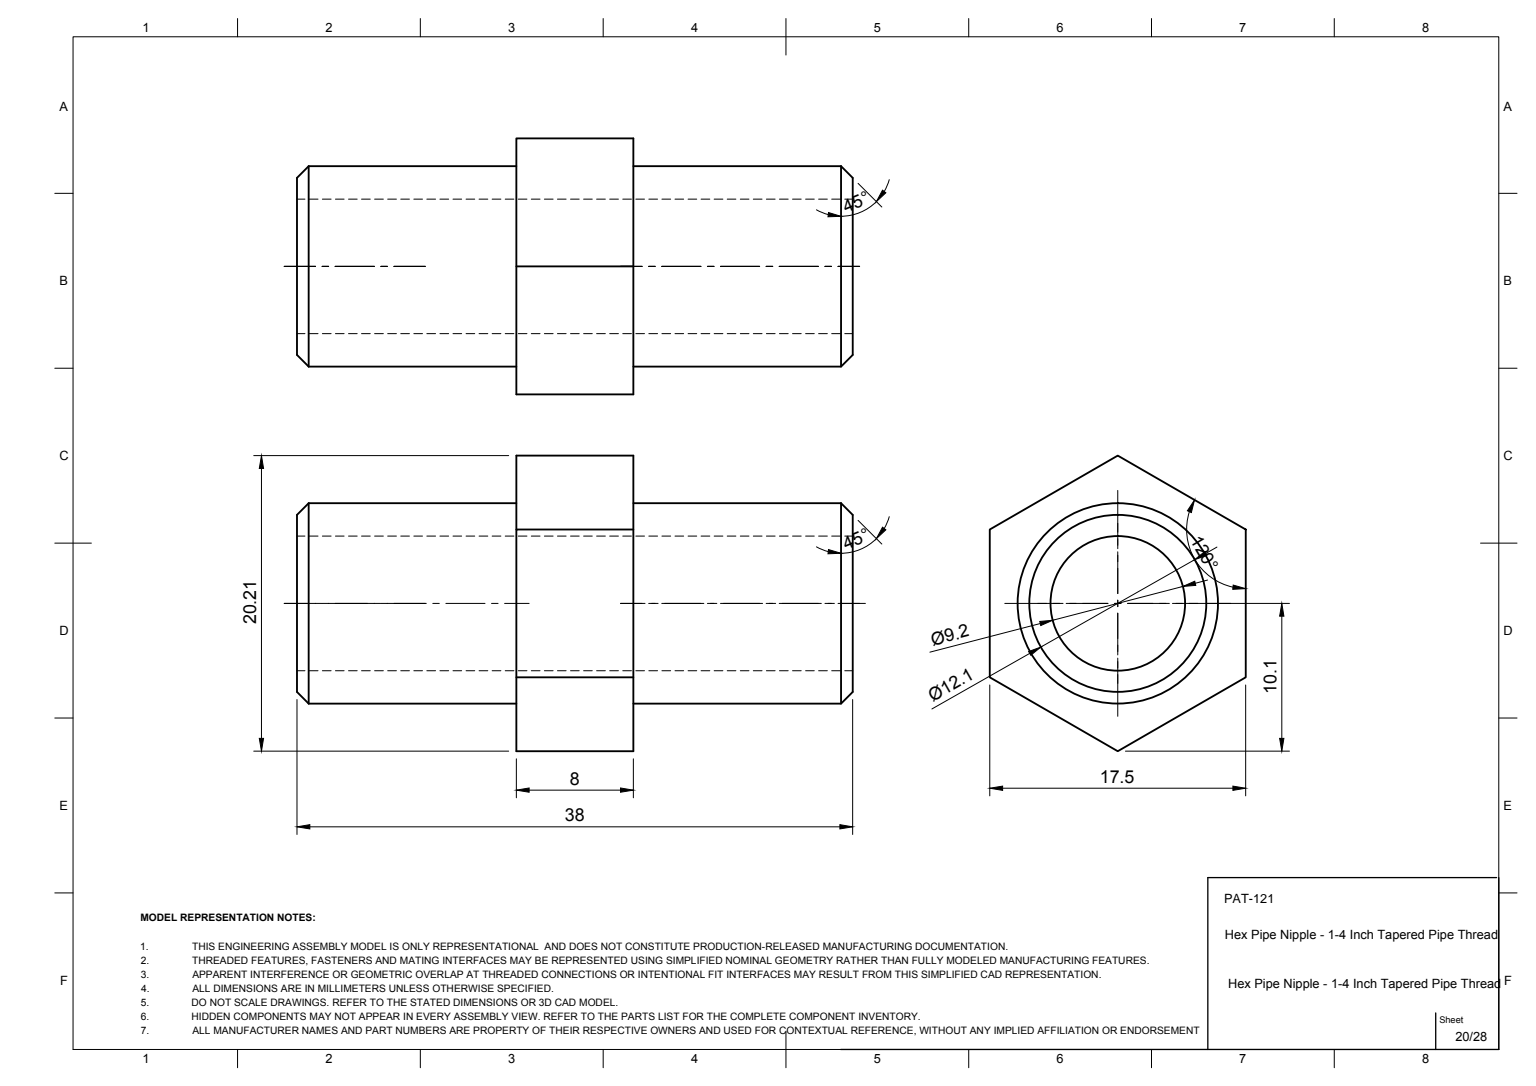
ISO-10303-21;
HEADER;
/* Generated by software containing ST-Developer
 * from STEP Tools, Inc. (www.steptools.com) 
 */

FILE_DESCRIPTION(
/* description */ ('Wall-mounted air drop station'),
/* implementation_level */ '2;1');

FILE_NAME(
/* name */ 'Hex Pipe Nipple - 1-4 Inch Tapered Pipe Thread.step',
/* time_stamp */ '2026-10-28T22:16:19-07:00',
/* author */ (''),
/* organization */ (''),
/* preprocessor_version */ 'ST-DEVELOPER v20.2',
/* originating_system */ 'Autodesk Translation Framework v15.17.0.0',
/* authorisation */ '');

FILE_SCHEMA (('AUTOMOTIVE_DESIGN { 1 0 10303 214 3 1 1 }'));
ENDSEC;

DATA;
#10=MECHANICAL_DESIGN_GEOMETRIC_PRESENTATION_REPRESENTATION('',(#365),#10517);
#279=CONICAL_SURFACE('',#6741,0.645,0.785398163397448);
#280=CONICAL_SURFACE('',#6744,0.645,0.785398163397448);
#307=SHAPE_REPRESENTATION_RELATIONSHIP('SRR','None',#10664,#336);
#336=ADVANCED_BREP_SHAPE_REPRESENTATION('',(#392),#10508);
#365=STYLED_ITEM('',(#10867),#392);
#392=MANIFOLD_SOLID_BREP('Body1',#5906);
#512=FACE_BOUND('',#1487,.T.);
#513=FACE_BOUND('',#1489,.T.);
#514=FACE_BOUND('',#1498,.T.);
#515=FACE_BOUND('',#1503,.T.);
#682=PLANE('',#6726);
#683=PLANE('',#6728);
#684=PLANE('',#6730);
#685=PLANE('',#6731);
#686=PLANE('',#6732);
#687=PLANE('',#6733);
#688=PLANE('',#6734);
#689=PLANE('',#6735);
#690=PLANE('',#6738);
#691=PLANE('',#6746);
#1018=FACE_OUTER_BOUND('',#1486,.T.);
#1019=FACE_OUTER_BOUND('',#1488,.T.);
#1020=FACE_OUTER_BOUND('',#1490,.T.);
#1021=FACE_OUTER_BOUND('',#1491,.T.);
#1022=FACE_OUTER_BOUND('',#1492,.T.);
#1023=FACE_OUTER_BOUND('',#1493,.T.);
#1024=FACE_OUTER_BOUND('',#1494,.T.);
#1025=FACE_OUTER_BOUND('',#1495,.T.);
#1026=FACE_OUTER_BOUND('',#1496,.T.);
#1027=FACE_OUTER_BOUND('',#1497,.T.);
#1028=FACE_OUTER_BOUND('',#1499,.T.);
#1029=FACE_OUTER_BOUND('',#1500,.T.);
#1030=FACE_OUTER_BOUND('',#1501,.T.);
#1031=FACE_OUTER_BOUND('',#1502,.T.);
#1032=FACE_OUTER_BOUND('',#1504,.T.);
#1486=EDGE_LOOP('',(#5049,#5050,#5051,#5052,#5053,#5054));
#1487=EDGE_LOOP('',(#5055));
#1488=EDGE_LOOP('',(#5056,#5057,#5058,#5059,#5060,#5061));
#1489=EDGE_LOOP('',(#5062));
#1490=EDGE_LOOP('',(#5063,#5064,#5065,#5066));
#1491=EDGE_LOOP('',(#5067,#5068,#5069,#5070));
#1492=EDGE_LOOP('',(#5071,#5072,#5073,#5074));
#1493=EDGE_LOOP('',(#5075,#5076,#5077,#5078));
#1494=EDGE_LOOP('',(#5079,#5080,#5081,#5082));
#1495=EDGE_LOOP('',(#5083,#5084,#5085,#5086));
#1496=EDGE_LOOP('',(#5087,#5088,#5089,#5090));
#1497=EDGE_LOOP('',(#5091));
#1498=EDGE_LOOP('',(#5092));
#1499=EDGE_LOOP('',(#5093,#5094,#5095,#5096));
#1500=EDGE_LOOP('',(#5097,#5098,#5099,#5100));
#1501=EDGE_LOOP('',(#5101,#5102,#5103,#5104));
#1502=EDGE_LOOP('',(#5105));
#1503=EDGE_LOOP('',(#5106));
#1504=EDGE_LOOP('',(#5107,#5108,#5109,#5110));
#1914=LINE('',#9974,#2378);
#1915=LINE('',#9976,#2379);
#1916=LINE('',#9978,#2380);
#1917=LINE('',#9980,#2381);
#1918=LINE('',#9982,#2382);
#1919=LINE('',#9983,#2383);
#1920=LINE('',#9989,#2384);
#1921=LINE('',#9991,#2385);
#1922=LINE('',#9993,#2386);
#1923=LINE('',#9995,#2387);
#1924=LINE('',#9997,#2388);
#1925=LINE('',#9998,#2389);
#1926=LINE('',#10002,#2390);
#1927=LINE('',#10003,#2391);
#1928=LINE('',#10005,#2392);
#1929=LINE('',#10007,#2393);
#1930=LINE('',#10009,#2394);
#1931=LINE('',#10011,#2395);
#1932=LINE('',#10015,#2396);
#1933=LINE('',#10023,#2397);
#1934=LINE('',#10027,#2398);
#1935=LINE('',#10031,#2399);
#1936=LINE('',#10036,#2400);
#2378=VECTOR('',#8230,1.);
#2379=VECTOR('',#8231,1.);
#2380=VECTOR('',#8232,1.);
#2381=VECTOR('',#8233,1.);
#2382=VECTOR('',#8234,1.);
#2383=VECTOR('',#8235,1.);
#2384=VECTOR('',#8240,1.);
#2385=VECTOR('',#8241,1.);
#2386=VECTOR('',#8242,1.);
#2387=VECTOR('',#8243,1.);
#2388=VECTOR('',#8244,1.);
#2389=VECTOR('',#8245,1.);
#2390=VECTOR('',#8250,1.);
#2391=VECTOR('',#8251,1.);
#2392=VECTOR('',#8254,1.);
#2393=VECTOR('',#8257,1.);
#2394=VECTOR('',#8260,1.);
#2395=VECTOR('',#8263,1.);
#2396=VECTOR('',#8268,0.685);
#2397=VECTOR('',#8279,0.645);
#2398=VECTOR('',#8284,0.685);
#2399=VECTOR('',#8289,0.645);
#2400=VECTOR('',#8296,0.46);
#2722=CIRCLE('',#6727,0.685);
#2723=CIRCLE('',#6729,0.685);
#2724=CIRCLE('',#6737,0.685);
#2725=CIRCLE('',#6739,0.605);
#2726=CIRCLE('',#6740,0.46);
#2727=CIRCLE('',#6743,0.685);
#2728=CIRCLE('',#6745,0.605);
#2729=CIRCLE('',#6747,0.46);
#3121=VERTEX_POINT('',#9972);
#3122=VERTEX_POINT('',#9973);
#3123=VERTEX_POINT('',#9975);
#3124=VERTEX_POINT('',#9977);
#3125=VERTEX_POINT('',#9979);
#3126=VERTEX_POINT('',#9981);
#3127=VERTEX_POINT('',#9984);
#3128=VERTEX_POINT('',#9987);
#3129=VERTEX_POINT('',#9988);
#3130=VERTEX_POINT('',#9990);
#3131=VERTEX_POINT('',#9992);
#3132=VERTEX_POINT('',#9994);
#3133=VERTEX_POINT('',#9996);
#3134=VERTEX_POINT('',#9999);
#3135=VERTEX_POINT('',#10014);
#3136=VERTEX_POINT('',#10018);
#3137=VERTEX_POINT('',#10020);
#3138=VERTEX_POINT('',#10025);
#3139=VERTEX_POINT('',#10029);
#3140=VERTEX_POINT('',#10033);
#3782=EDGE_CURVE('',#3121,#3122,#1914,.T.);
#3783=EDGE_CURVE('',#3122,#3123,#1915,.T.);
#3784=EDGE_CURVE('',#3123,#3124,#1916,.T.);
#3785=EDGE_CURVE('',#3124,#3125,#1917,.T.);
#3786=EDGE_CURVE('',#3125,#3126,#1918,.T.);
#3787=EDGE_CURVE('',#3126,#3121,#1919,.T.);
#3788=EDGE_CURVE('',#3127,#3127,#2722,.T.);
#3789=EDGE_CURVE('',#3128,#3129,#1920,.T.);
#3790=EDGE_CURVE('',#3129,#3130,#1921,.T.);
#3791=EDGE_CURVE('',#3130,#3131,#1922,.T.);
#3792=EDGE_CURVE('',#3131,#3132,#1923,.T.);
#3793=EDGE_CURVE('',#3132,#3133,#1924,.T.);
#3794=EDGE_CURVE('',#3133,#3128,#1925,.T.);
#3795=EDGE_CURVE('',#3134,#3134,#2723,.T.);
#3796=EDGE_CURVE('',#3128,#3122,#1926,.T.);
#3797=EDGE_CURVE('',#3123,#3133,#1927,.T.);
#3798=EDGE_CURVE('',#3124,#3132,#1928,.T.);
#3799=EDGE_CURVE('',#3125,#3131,#1929,.T.);
#3800=EDGE_CURVE('',#3126,#3130,#1930,.T.);
#3801=EDGE_CURVE('',#3121,#3129,#1931,.T.);
#3802=EDGE_CURVE('',#3134,#3135,#1932,.T.);
#3803=EDGE_CURVE('',#3135,#3135,#2724,.T.);
#3804=EDGE_CURVE('',#3136,#3136,#2725,.T.);
#3805=EDGE_CURVE('',#3137,#3137,#2726,.T.);
#3806=EDGE_CURVE('',#3135,#3136,#1933,.T.);
#3807=EDGE_CURVE('',#3138,#3138,#2727,.T.);
#3808=EDGE_CURVE('',#3138,#3127,#1934,.T.);
#3809=EDGE_CURVE('',#3139,#3139,#2728,.T.);
#3810=EDGE_CURVE('',#3139,#3138,#1935,.T.);
#3811=EDGE_CURVE('',#3140,#3140,#2729,.T.);
#3812=EDGE_CURVE('',#3140,#3137,#1936,.T.);
#5049=ORIENTED_EDGE('',*,*,#3782,.T.);
#5050=ORIENTED_EDGE('',*,*,#3783,.T.);
#5051=ORIENTED_EDGE('',*,*,#3784,.T.);
#5052=ORIENTED_EDGE('',*,*,#3785,.T.);
#5053=ORIENTED_EDGE('',*,*,#3786,.T.);
#5054=ORIENTED_EDGE('',*,*,#3787,.T.);
#5055=ORIENTED_EDGE('',*,*,#3788,.F.);
#5056=ORIENTED_EDGE('',*,*,#3789,.T.);
#5057=ORIENTED_EDGE('',*,*,#3790,.T.);
#5058=ORIENTED_EDGE('',*,*,#3791,.T.);
#5059=ORIENTED_EDGE('',*,*,#3792,.T.);
#5060=ORIENTED_EDGE('',*,*,#3793,.T.);
#5061=ORIENTED_EDGE('',*,*,#3794,.T.);
#5062=ORIENTED_EDGE('',*,*,#3795,.F.);
#5063=ORIENTED_EDGE('',*,*,#3796,.F.);
#5064=ORIENTED_EDGE('',*,*,#3794,.F.);
#5065=ORIENTED_EDGE('',*,*,#3797,.F.);
#5066=ORIENTED_EDGE('',*,*,#3783,.F.);
#5067=ORIENTED_EDGE('',*,*,#3797,.T.);
#5068=ORIENTED_EDGE('',*,*,#3793,.F.);
#5069=ORIENTED_EDGE('',*,*,#3798,.F.);
#5070=ORIENTED_EDGE('',*,*,#3784,.F.);
#5071=ORIENTED_EDGE('',*,*,#3798,.T.);
#5072=ORIENTED_EDGE('',*,*,#3792,.F.);
#5073=ORIENTED_EDGE('',*,*,#3799,.F.);
#5074=ORIENTED_EDGE('',*,*,#3785,.F.);
#5075=ORIENTED_EDGE('',*,*,#3799,.T.);
#5076=ORIENTED_EDGE('',*,*,#3791,.F.);
#5077=ORIENTED_EDGE('',*,*,#3800,.F.);
#5078=ORIENTED_EDGE('',*,*,#3786,.F.);
#5079=ORIENTED_EDGE('',*,*,#3800,.T.);
#5080=ORIENTED_EDGE('',*,*,#3790,.F.);
#5081=ORIENTED_EDGE('',*,*,#3801,.F.);
#5082=ORIENTED_EDGE('',*,*,#3787,.F.);
#5083=ORIENTED_EDGE('',*,*,#3801,.T.);
#5084=ORIENTED_EDGE('',*,*,#3789,.F.);
#5085=ORIENTED_EDGE('',*,*,#3796,.T.);
#5086=ORIENTED_EDGE('',*,*,#3782,.F.);
#5087=ORIENTED_EDGE('',*,*,#3795,.T.);
#5088=ORIENTED_EDGE('',*,*,#3802,.T.);
#5089=ORIENTED_EDGE('',*,*,#3803,.T.);
#5090=ORIENTED_EDGE('',*,*,#3802,.F.);
#5091=ORIENTED_EDGE('',*,*,#3804,.F.);
#5092=ORIENTED_EDGE('',*,*,#3805,.T.);
#5093=ORIENTED_EDGE('',*,*,#3803,.F.);
#5094=ORIENTED_EDGE('',*,*,#3806,.T.);
#5095=ORIENTED_EDGE('',*,*,#3804,.T.);
#5096=ORIENTED_EDGE('',*,*,#3806,.F.);
#5097=ORIENTED_EDGE('',*,*,#3807,.F.);
#5098=ORIENTED_EDGE('',*,*,#3808,.T.);
#5099=ORIENTED_EDGE('',*,*,#3788,.T.);
#5100=ORIENTED_EDGE('',*,*,#3808,.F.);
#5101=ORIENTED_EDGE('',*,*,#3809,.F.);
#5102=ORIENTED_EDGE('',*,*,#3810,.T.);
#5103=ORIENTED_EDGE('',*,*,#3807,.T.);
#5104=ORIENTED_EDGE('',*,*,#3810,.F.);
#5105=ORIENTED_EDGE('',*,*,#3809,.T.);
#5106=ORIENTED_EDGE('',*,*,#3811,.F.);
#5107=ORIENTED_EDGE('',*,*,#3811,.T.);
#5108=ORIENTED_EDGE('',*,*,#3812,.T.);
#5109=ORIENTED_EDGE('',*,*,#3805,.F.);
#5110=ORIENTED_EDGE('',*,*,#3812,.F.);
#5517=CYLINDRICAL_SURFACE('',#6736,0.685);
#5518=CYLINDRICAL_SURFACE('',#6742,0.685);
#5519=CYLINDRICAL_SURFACE('',#6748,0.46);
#5791=ADVANCED_FACE('',(#1018,#512),#682,.F.);
#5792=ADVANCED_FACE('',(#1019,#513),#683,.T.);
#5793=ADVANCED_FACE('',(#1020),#684,.T.);
#5794=ADVANCED_FACE('',(#1021),#685,.T.);
#5795=ADVANCED_FACE('',(#1022),#686,.T.);
#5796=ADVANCED_FACE('',(#1023),#687,.T.);
#5797=ADVANCED_FACE('',(#1024),#688,.T.);
#5798=ADVANCED_FACE('',(#1025),#689,.T.);
#5799=ADVANCED_FACE('',(#1026),#5517,.T.);
#5800=ADVANCED_FACE('',(#1027,#514),#690,.T.);
#5801=ADVANCED_FACE('',(#1028),#279,.T.);
#5802=ADVANCED_FACE('',(#1029),#5518,.T.);
#5803=ADVANCED_FACE('',(#1030),#280,.T.);
#5804=ADVANCED_FACE('',(#1031,#515),#691,.T.);
#5805=ADVANCED_FACE('',(#1032),#5519,.F.);
#5906=CLOSED_SHELL('',(#5791,#5792,#5793,#5794,#5795,#5796,#5797,#5798,
#5799,#5800,#5801,#5802,#5803,#5804,#5805));
#6725=AXIS2_PLACEMENT_3D('',#9970,#8226,#8227);
#6726=AXIS2_PLACEMENT_3D('',#9971,#8228,#8229);
#6727=AXIS2_PLACEMENT_3D('',#9985,#8236,#8237);
#6728=AXIS2_PLACEMENT_3D('',#9986,#8238,#8239);
#6729=AXIS2_PLACEMENT_3D('',#10000,#8246,#8247);
#6730=AXIS2_PLACEMENT_3D('',#10001,#8248,#8249);
#6731=AXIS2_PLACEMENT_3D('',#10004,#8252,#8253);
#6732=AXIS2_PLACEMENT_3D('',#10006,#8255,#8256);
#6733=AXIS2_PLACEMENT_3D('',#10008,#8258,#8259);
#6734=AXIS2_PLACEMENT_3D('',#10010,#8261,#8262);
#6735=AXIS2_PLACEMENT_3D('',#10012,#8264,#8265);
#6736=AXIS2_PLACEMENT_3D('',#10013,#8266,#8267);
#6737=AXIS2_PLACEMENT_3D('',#10016,#8269,#8270);
#6738=AXIS2_PLACEMENT_3D('',#10017,#8271,#8272);
#6739=AXIS2_PLACEMENT_3D('',#10019,#8273,#8274);
#6740=AXIS2_PLACEMENT_3D('',#10021,#8275,#8276);
#6741=AXIS2_PLACEMENT_3D('',#10022,#8277,#8278);
#6742=AXIS2_PLACEMENT_3D('',#10024,#8280,#8281);
#6743=AXIS2_PLACEMENT_3D('',#10026,#8282,#8283);
#6744=AXIS2_PLACEMENT_3D('',#10028,#8285,#8286);
#6745=AXIS2_PLACEMENT_3D('',#10030,#8287,#8288);
#6746=AXIS2_PLACEMENT_3D('',#10032,#8290,#8291);
#6747=AXIS2_PLACEMENT_3D('',#10034,#8292,#8293);
#6748=AXIS2_PLACEMENT_3D('',#10035,#8294,#8295);
#8226=DIRECTION('axis',(0.,0.,1.));
#8227=DIRECTION('refdir',(1.,0.,0.));
#8228=DIRECTION('center_axis',(0.,1.,0.));
#8229=DIRECTION('ref_axis',(1.,0.,0.));
#8230=DIRECTION('',(-0.5,0.,0.866025403784439));
#8231=DIRECTION('',(-1.,0.,-3.29650746237182E-16));
#8232=DIRECTION('',(-0.5,0.,-0.866025403784439));
#8233=DIRECTION('',(0.5,0.,-0.866025403784438));
#8234=DIRECTION('',(1.,0.,0.));
#8235=DIRECTION('',(0.5,0.,0.866025403784439));
#8236=DIRECTION('center_axis',(0.,-1.,0.));
#8237=DIRECTION('ref_axis',(1.,0.,0.));
#8238=DIRECTION('center_axis',(0.,1.,0.));
#8239=DIRECTION('ref_axis',(1.,0.,0.));
#8240=DIRECTION('',(0.5,0.,-0.866025403784439));
#8241=DIRECTION('',(-0.5,0.,-0.866025403784439));
#8242=DIRECTION('',(-1.,0.,0.));
#8243=DIRECTION('',(-0.5,0.,0.866025403784438));
#8244=DIRECTION('',(0.5,0.,0.866025403784439));
#8245=DIRECTION('',(1.,0.,3.29650746237182E-16));
#8246=DIRECTION('center_axis',(0.,1.,0.));
#8247=DIRECTION('ref_axis',(1.,0.,0.));
#8248=DIRECTION('center_axis',(-3.29650746237182E-16,0.,1.));
#8249=DIRECTION('ref_axis',(1.,0.,3.29650746237182E-16));
#8250=DIRECTION('',(0.,-1.,0.));
#8251=DIRECTION('',(0.,1.,0.));
#8252=DIRECTION('center_axis',(-0.866025403784439,0.,0.5));
#8253=DIRECTION('ref_axis',(0.5,0.,0.866025403784439));
#8254=DIRECTION('',(0.,1.,0.));
#8255=DIRECTION('center_axis',(-0.866025403784439,0.,-0.5));
#8256=DIRECTION('ref_axis',(-0.5,0.,0.866025403784439));
#8257=DIRECTION('',(0.,1.,0.));
#8258=DIRECTION('center_axis',(0.,0.,-1.));
#8259=DIRECTION('ref_axis',(-1.,0.,0.));
#8260=DIRECTION('',(0.,1.,0.));
#8261=DIRECTION('center_axis',(0.866025403784439,0.,-0.5));
#8262=DIRECTION('ref_axis',(-0.5,0.,-0.866025403784439));
#8263=DIRECTION('',(0.,1.,0.));
#8264=DIRECTION('center_axis',(0.866025403784439,0.,0.5));
#8265=DIRECTION('ref_axis',(0.5,0.,-0.866025403784439));
#8266=DIRECTION('center_axis',(0.,-1.,0.));
#8267=DIRECTION('ref_axis',(1.,0.,0.));
#8268=DIRECTION('',(0.,1.,0.));
#8269=DIRECTION('center_axis',(0.,-1.,0.));
#8270=DIRECTION('ref_axis',(1.,0.,0.));
#8271=DIRECTION('center_axis',(0.,1.,0.));
#8272=DIRECTION('ref_axis',(0.,0.,1.));
#8273=DIRECTION('center_axis',(0.,-1.,0.));
#8274=DIRECTION('ref_axis',(1.,0.,0.));
#8275=DIRECTION('center_axis',(0.,-1.,0.));
#8276=DIRECTION('ref_axis',(1.,0.,0.));
#8277=DIRECTION('center_axis',(0.,-1.,0.));
#8278=DIRECTION('ref_axis',(1.,0.,0.));
#8279=DIRECTION('',(0.707106781186547,0.707106781186548,8.65956056235493E-17));
#8280=DIRECTION('center_axis',(0.,-1.,0.));
#8281=DIRECTION('ref_axis',(1.,0.,0.));
#8282=DIRECTION('center_axis',(0.,-1.,0.));
#8283=DIRECTION('ref_axis',(1.,0.,0.));
#8284=DIRECTION('',(0.,1.,0.));
#8285=DIRECTION('center_axis',(0.,1.,0.));
#8286=DIRECTION('ref_axis',(1.,0.,0.));
#8287=DIRECTION('center_axis',(0.,-1.,0.));
#8288=DIRECTION('ref_axis',(1.,0.,0.));
#8289=DIRECTION('',(-0.707106781186547,0.707106781186548,-8.65956056235493E-17));
#8290=DIRECTION('center_axis',(0.,-1.,0.));
#8291=DIRECTION('ref_axis',(0.,0.,-1.));
#8292=DIRECTION('center_axis',(0.,-1.,0.));
#8293=DIRECTION('ref_axis',(1.,0.,0.));
#8294=DIRECTION('center_axis',(0.,-1.,0.));
#8295=DIRECTION('ref_axis',(1.,0.,0.));
#8296=DIRECTION('',(0.,1.,0.));
#9970=CARTESIAN_POINT('',(0.,0.,0.));
#9971=CARTESIAN_POINT('Origin',(0.,-0.4,0.));
#9972=CARTESIAN_POINT('',(1.01036297108185,-0.4,0.));
#9973=CARTESIAN_POINT('',(0.505181485540923,-0.4,0.875));
#9974=CARTESIAN_POINT('',(0.505181485540923,-0.4,0.875));
#9975=CARTESIAN_POINT('',(-0.505181485540923,-0.4,0.875));
#9976=CARTESIAN_POINT('',(-0.505181485540923,-0.4,0.875));
#9977=CARTESIAN_POINT('',(-1.01036297108185,-0.4,-1.23733777851239E-16));
#9978=CARTESIAN_POINT('',(-1.01036297108185,-0.4,-1.23733777851239E-16));
#9979=CARTESIAN_POINT('',(-0.505181485540922,-0.4,-0.875));
#9980=CARTESIAN_POINT('',(-0.505181485540922,-0.4,-0.875));
#9981=CARTESIAN_POINT('',(0.505181485540923,-0.4,-0.875));
#9982=CARTESIAN_POINT('',(0.505181485540923,-0.4,-0.875));
#9983=CARTESIAN_POINT('',(1.01036297108185,-0.4,0.));
#9984=CARTESIAN_POINT('',(-0.685,-0.4,-8.38883057415937E-17));
#9985=CARTESIAN_POINT('Origin',(0.,-0.4,0.));
#9986=CARTESIAN_POINT('Origin',(0.,0.4,0.));
#9987=CARTESIAN_POINT('',(0.505181485540923,0.4,0.875));
#9988=CARTESIAN_POINT('',(1.01036297108185,0.4,0.));
#9989=CARTESIAN_POINT('',(0.505181485540923,0.4,0.875));
#9990=CARTESIAN_POINT('',(0.505181485540923,0.4,-0.875));
#9991=CARTESIAN_POINT('',(1.01036297108185,0.4,0.));
#9992=CARTESIAN_POINT('',(-0.505181485540922,0.4,-0.875));
#9993=CARTESIAN_POINT('',(0.505181485540923,0.4,-0.875));
#9994=CARTESIAN_POINT('',(-1.01036297108185,0.4,-1.23733777851239E-16));
#9995=CARTESIAN_POINT('',(-0.505181485540922,0.4,-0.875));
#9996=CARTESIAN_POINT('',(-0.505181485540923,0.4,0.875));
#9997=CARTESIAN_POINT('',(-1.01036297108185,0.4,-1.23733777851239E-16));
#9998=CARTESIAN_POINT('',(-0.505181485540923,0.4,0.875));
#9999=CARTESIAN_POINT('',(-0.685,0.4,8.38883057415937E-17));
#10000=CARTESIAN_POINT('Origin',(0.,0.4,0.));
#10001=CARTESIAN_POINT('Origin',(-0.505181485540923,0.,0.875));
#10002=CARTESIAN_POINT('',(0.505181485540923,0.,0.875));
#10003=CARTESIAN_POINT('',(-0.505181485540923,0.,0.875));
#10004=CARTESIAN_POINT('Origin',(-1.01036297108185,0.,-1.23733777851239E-16));
#10005=CARTESIAN_POINT('',(-1.01036297108185,0.,-1.23733777851239E-16));
#10006=CARTESIAN_POINT('Origin',(-0.505181485540922,0.,-0.875));
#10007=CARTESIAN_POINT('',(-0.505181485540922,0.,-0.875));
#10008=CARTESIAN_POINT('Origin',(0.505181485540923,0.,-0.875));
#10009=CARTESIAN_POINT('',(0.505181485540923,0.,-0.875));
#10010=CARTESIAN_POINT('Origin',(1.01036297108185,0.,0.));
#10011=CARTESIAN_POINT('',(1.01036297108185,0.,0.));
#10012=CARTESIAN_POINT('Origin',(0.505181485540923,0.,0.875));
#10013=CARTESIAN_POINT('Origin',(0.,0.,0.));
#10014=CARTESIAN_POINT('',(-0.685,1.82,-8.38883057415937E-17));
#10015=CARTESIAN_POINT('',(-0.685,0.,-8.38883057415937E-17));
#10016=CARTESIAN_POINT('Origin',(0.,1.82,0.));
#10017=CARTESIAN_POINT('Origin',(0.605,1.9,0.));
#10018=CARTESIAN_POINT('',(-0.605,1.9,-7.40911313484149E-17));
#10019=CARTESIAN_POINT('Origin',(0.,1.9,0.));
#10020=CARTESIAN_POINT('',(-0.46,1.9,-5.63337527607782E-17));
#10021=CARTESIAN_POINT('Origin',(0.,1.9,0.));
#10022=CARTESIAN_POINT('Origin',(0.,1.86,0.));
#10023=CARTESIAN_POINT('',(-0.645,1.86,-7.89897185450043E-17));
#10024=CARTESIAN_POINT('Origin',(0.,0.,0.));
#10025=CARTESIAN_POINT('',(-0.685,-1.82,-8.38883057415937E-17));
#10026=CARTESIAN_POINT('Origin',(0.,-1.82,0.));
#10027=CARTESIAN_POINT('',(-0.685,0.,-8.38883057415937E-17));
#10028=CARTESIAN_POINT('Origin',(0.,-1.86,0.));
#10029=CARTESIAN_POINT('',(-0.605,-1.9,-7.40911313484149E-17));
#10030=CARTESIAN_POINT('Origin',(0.,-1.9,0.));
#10031=CARTESIAN_POINT('',(-0.645,-1.86,-7.89897185450043E-17));
#10032=CARTESIAN_POINT('Origin',(0.46,-1.9,0.));
#10033=CARTESIAN_POINT('',(-0.46,-1.9,-5.63337527607782E-17));
#10034=CARTESIAN_POINT('Origin',(0.,-1.9,0.));
#10035=CARTESIAN_POINT('Origin',(0.,0.,0.));
#10036=CARTESIAN_POINT('',(-0.46,0.,-5.63337527607782E-17));
#10475=UNCERTAINTY_MEASURE_WITH_UNIT(LENGTH_MEASURE(0.001),#10518,
'DISTANCE_ACCURACY_VALUE',
'Maximum model space distance between geometric entities at asserted c
onnectivities');
#10484=UNCERTAINTY_MEASURE_WITH_UNIT(LENGTH_MEASURE(0.001),#10518,
'DISTANCE_ACCURACY_VALUE',
'Maximum model space distance between geometric entities at asserted c
onnectivities');
#10508=(
GEOMETRIC_REPRESENTATION_CONTEXT(3)
GLOBAL_UNCERTAINTY_ASSIGNED_CONTEXT((#10475))
GLOBAL_UNIT_ASSIGNED_CONTEXT((#10518,#10520,#10521))
REPRESENTATION_CONTEXT('','3D')
);
#10517=(
GEOMETRIC_REPRESENTATION_CONTEXT(3)
GLOBAL_UNCERTAINTY_ASSIGNED_CONTEXT((#10484))
GLOBAL_UNIT_ASSIGNED_CONTEXT((#10518,#10520,#10521))
REPRESENTATION_CONTEXT('','3D')
);
#10518=(
LENGTH_UNIT()
NAMED_UNIT(*)
SI_UNIT(.CENTI.,.METRE.)
);
#10520=(
NAMED_UNIT(*)
PLANE_ANGLE_UNIT()
SI_UNIT($,.RADIAN.)
);
#10521=(
NAMED_UNIT(*)
SI_UNIT($,.STERADIAN.)
SOLID_ANGLE_UNIT()
);
#10545=SHAPE_DEFINITION_REPRESENTATION(#10577,#10664);
#10577=PRODUCT_DEFINITION_SHAPE('',$,#10697);
#10664=SHAPE_REPRESENTATION('',(#6725),#10508);
#10673=PRODUCT_DEFINITION_CONTEXT('part definition',#10771,'design');
#10697=PRODUCT_DEFINITION(
'Hex Pipe Nipple - 1-4 Inch Tapered Pipe Thread',
'Hex Pipe Nipple - 1-4 Inch Tapered Pipe Thread',#10729,#10673);
#10729=PRODUCT_DEFINITION_FORMATION('',$,#10796);
#10771=APPLICATION_CONTEXT(
'Core Data for Automotive Mechanical Design Process');
#10772=PRODUCT_CONTEXT('part definition',#10771,'mechanical');
#10796=PRODUCT('Hex Pipe Nipple - 1-4 Inch Tapered Pipe Thread',
'Hex Pipe Nipple - 1-4 Inch Tapered Pipe Thread',
'Hex Pipe Nipple - 1-4 Inch Tapered Pipe Thread',(#10772));
#10861=COLOUR_RGB('Sky Blue',0.24,0.69,0.87);
#10862=FILL_AREA_STYLE_COLOUR('',#10861);
#10863=FILL_AREA_STYLE('',(#10862));
#10864=SURFACE_STYLE_FILL_AREA(#10863);
#10865=SURFACE_SIDE_STYLE('',(#10864));
#10866=SURFACE_STYLE_USAGE(.BOTH.,#10865);
#10867=PRESENTATION_STYLE_ASSIGNMENT((#10866));
ENDSEC;
END-ISO-10303-21;
